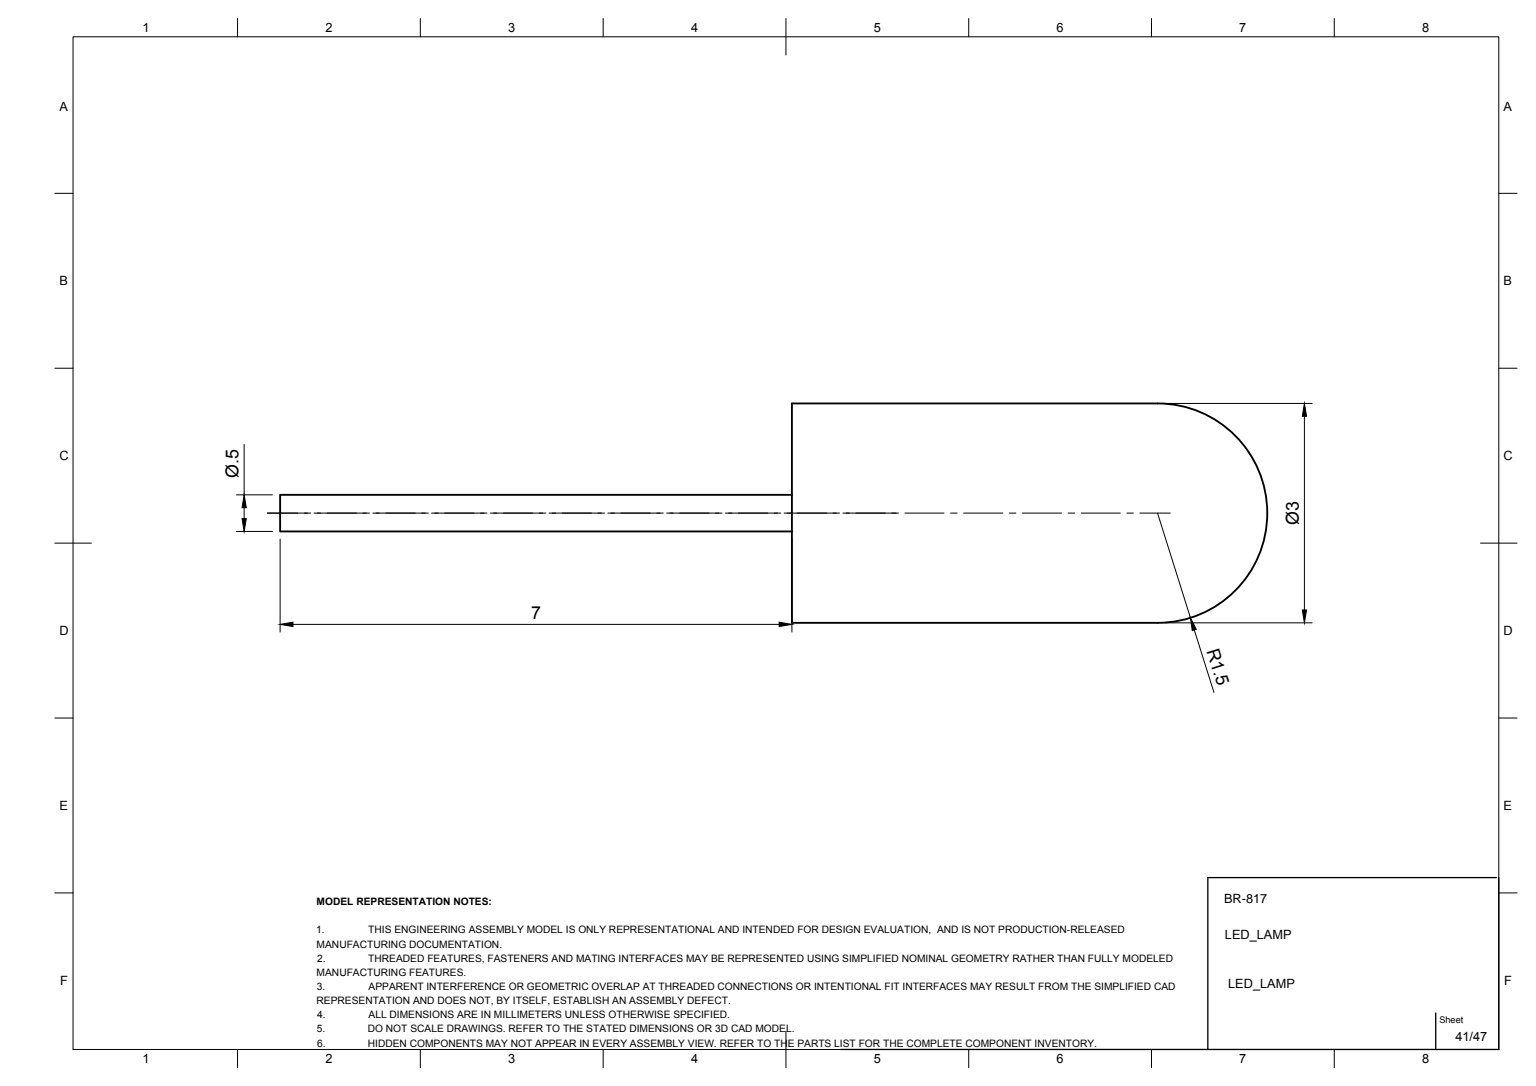
ISO-10303-21;
HEADER;
FILE_DESCRIPTION((''),'2;1');
FILE_NAME('LED_LAMP.step','2026-10-01T22:07:29-07:00',(''),(''),'','','');
FILE_SCHEMA (('AUTOMOTIVE_DESIGN { 1 0 10303 214 3 1 1 }'));
ENDSEC;
DATA;
#10=MECHANICAL_DESIGN_GEOMETRIC_PRESENTATION_REPRESENTATION('',(#572,#573,#574),#15484);
#291=SPHERICAL_SURFACE('',#9810,0.15) ;
#292=SPHERICAL_SURFACE('',#9813,0.15) ;
#501=SHAPE_REPRESENTATION_RELATIONSHIP('SRR','None',#15652,#536) ;
#536=ADVANCED_BREP_SHAPE_REPRESENTATION('',(#613,#614,#615),#15476) ;
#572=STYLED_ITEM('',(#15841),#613) ;
#573=STYLED_ITEM('',(#15842),#614) ;
#574=STYLED_ITEM('',(#15842),#615) ;
#613=MANIFOLD_SOLID_BREP('LED_BODY',#8283) ;
#614=MANIFOLD_SOLID_BREP('LED_LEADS',#8284) ;
#615=MANIFOLD_SOLID_BREP('LED_LEADS',#8285) ;
#795=CYLINDRICAL_SURFACE('',#9815,0.15) ;
#796=CYLINDRICAL_SURFACE('',#9818,0.025) ;
#797=CYLINDRICAL_SURFACE('',#9823,0.025) ;
#1329=CIRCLE('',#9811,0.15) ;
#1330=CIRCLE('',#9812,0.15) ;
#1331=CIRCLE('',#9814,0.15) ;
#1332=CIRCLE('',#9816,0.15) ;
#1333=CIRCLE('',#9819,0.025) ;
#1334=CIRCLE('',#9820,0.025) ;
#1335=CIRCLE('',#9824,0.025) ;
#1336=CIRCLE('',#9825,0.025) ;
#1812=FACE_OUTER_BOUND('',#2383,.T.) ;
#1813=FACE_OUTER_BOUND('',#2384,.T.) ;
#1814=FACE_OUTER_BOUND('',#2385,.T.) ;
#1815=FACE_OUTER_BOUND('',#2386,.T.) ;
#1816=FACE_OUTER_BOUND('',#2387,.T.) ;
#1817=FACE_OUTER_BOUND('',#2388,.T.) ;
#1818=FACE_OUTER_BOUND('',#2389,.T.) ;
#1819=FACE_OUTER_BOUND('',#2390,.T.) ;
#1820=FACE_OUTER_BOUND('',#2391,.T.) ;
#1821=FACE_OUTER_BOUND('',#2392,.T.) ;
#2383=EDGE_LOOP('',(#7377,#7378)) ;
#2384=EDGE_LOOP('',(#7379,#7380)) ;
#2385=EDGE_LOOP('',(#7381,#7382,#7383,#7384,#7385)) ;
#2386=EDGE_LOOP('',(#7386)) ;
#2387=EDGE_LOOP('',(#7387,#7388,#7389,#7390)) ;
#2388=EDGE_LOOP('',(#7391)) ;
#2389=EDGE_LOOP('',(#7392)) ;
#2390=EDGE_LOOP('',(#7393,#7394,#7395,#7396)) ;
#2391=EDGE_LOOP('',(#7397)) ;
#2392=EDGE_LOOP('',(#7398)) ;
#2870=LINE('',#15197,#3344) ;
#2871=LINE('',#15203,#3345) ;
#2872=LINE('',#15211,#3346) ;
#3344=VECTOR('',#12625,0.15) ;
#3345=VECTOR('',#12632,0.025) ;
#3346=VECTOR('',#12643,0.025) ;
#4088=VERTEX_POINT('',#15188) ;
#4089=VERTEX_POINT('',#15189) ;
#4090=VERTEX_POINT('',#15195) ;
#4091=VERTEX_POINT('',#15200) ;
#4092=VERTEX_POINT('',#15202) ;
#4093=VERTEX_POINT('',#15208) ;
#4094=VERTEX_POINT('',#15210) ;
#5193=EDGE_CURVE('',#4088,#4089,#1329,.T.) ;
#5194=EDGE_CURVE('',#4088,#4089,#1330,.T.) ;
#5195=EDGE_CURVE('',#4089,#4088,#1331,.T.) ;
#5196=EDGE_CURVE('',#4090,#4090,#1332,.T.) ;
#5197=EDGE_CURVE('',#4090,#4088,#2870,.T.) ;
#5198=EDGE_CURVE('',#4091,#4091,#1333,.T.) ;
#5199=EDGE_CURVE('',#4091,#4092,#2871,.T.) ;
#5200=EDGE_CURVE('',#4092,#4092,#1334,.T.) ;
#5201=EDGE_CURVE('',#4093,#4093,#1335,.T.) ;
#5202=EDGE_CURVE('',#4093,#4094,#2872,.T.) ;
#5203=EDGE_CURVE('',#4094,#4094,#1336,.T.) ;
#7377=ORIENTED_EDGE('',*,*,#5193,.F.) ;
#7378=ORIENTED_EDGE('',*,*,#5194,.T.) ;
#7379=ORIENTED_EDGE('',*,*,#5193,.T.) ;
#7380=ORIENTED_EDGE('',*,*,#5195,.T.) ;
#7381=ORIENTED_EDGE('',*,*,#5196,.F.) ;
#7382=ORIENTED_EDGE('',*,*,#5197,.T.) ;
#7383=ORIENTED_EDGE('',*,*,#5195,.F.) ;
#7384=ORIENTED_EDGE('',*,*,#5194,.F.) ;
#7385=ORIENTED_EDGE('',*,*,#5197,.F.) ;
#7386=ORIENTED_EDGE('',*,*,#5196,.T.) ;
#7387=ORIENTED_EDGE('',*,*,#5198,.F.) ;
#7388=ORIENTED_EDGE('',*,*,#5199,.T.) ;
#7389=ORIENTED_EDGE('',*,*,#5200,.F.) ;
#7390=ORIENTED_EDGE('',*,*,#5199,.F.) ;
#7391=ORIENTED_EDGE('',*,*,#5200,.T.) ;
#7392=ORIENTED_EDGE('',*,*,#5198,.T.) ;
#7393=ORIENTED_EDGE('',*,*,#5201,.F.) ;
#7394=ORIENTED_EDGE('',*,*,#5202,.T.) ;
#7395=ORIENTED_EDGE('',*,*,#5203,.F.) ;
#7396=ORIENTED_EDGE('',*,*,#5202,.F.) ;
#7397=ORIENTED_EDGE('',*,*,#5203,.T.) ;
#7398=ORIENTED_EDGE('',*,*,#5201,.T.) ;
#7716=PLANE('',#9817) ;
#7717=PLANE('',#9821) ;
#7718=PLANE('',#9822) ;
#7719=PLANE('',#9826) ;
#7720=PLANE('',#9827) ;
#8199=ADVANCED_FACE('',(#1812),#291,.T.) ;
#8200=ADVANCED_FACE('',(#1813),#292,.T.) ;
#8201=ADVANCED_FACE('',(#1814),#795,.T.) ;
#8202=ADVANCED_FACE('',(#1815),#7716,.T.) ;
#8203=ADVANCED_FACE('',(#1816),#796,.T.) ;
#8204=ADVANCED_FACE('',(#1817),#7717,.T.) ;
#8205=ADVANCED_FACE('',(#1818),#7718,.T.) ;
#8206=ADVANCED_FACE('',(#1819),#797,.T.) ;
#8207=ADVANCED_FACE('',(#1820),#7719,.T.) ;
#8208=ADVANCED_FACE('',(#1821),#7720,.T.) ;
#8283=CLOSED_SHELL('',(#8199,#8200,#8201,#8202)) ;
#8284=CLOSED_SHELL('',(#8203,#8204,#8205)) ;
#8285=CLOSED_SHELL('',(#8206,#8207,#8208)) ;
#9809=AXIS2_PLACEMENT_3D('',#15186,#12609,#12610) ;
#9810=AXIS2_PLACEMENT_3D('',#15187,#12611,#12612) ;
#9811=AXIS2_PLACEMENT_3D('',#15190,#12613,#12614) ;
#9812=AXIS2_PLACEMENT_3D('',#15191,#12615,#12616) ;
#9813=AXIS2_PLACEMENT_3D('',#15192,#12617,#12618) ;
#9814=AXIS2_PLACEMENT_3D('',#15193,#12619,#12620) ;
#9815=AXIS2_PLACEMENT_3D('',#15194,#12621,#12622) ;
#9816=AXIS2_PLACEMENT_3D('',#15196,#12623,#12624) ;
#9817=AXIS2_PLACEMENT_3D('',#15198,#12626,#12627) ;
#9818=AXIS2_PLACEMENT_3D('',#15199,#12628,#12629) ;
#9819=AXIS2_PLACEMENT_3D('',#15201,#12630,#12631) ;
#9820=AXIS2_PLACEMENT_3D('',#15204,#12633,#12634) ;
#9821=AXIS2_PLACEMENT_3D('',#15205,#12635,#12636) ;
#9822=AXIS2_PLACEMENT_3D('',#15206,#12637,#12638) ;
#9823=AXIS2_PLACEMENT_3D('',#15207,#12639,#12640) ;
#9824=AXIS2_PLACEMENT_3D('',#15209,#12641,#12642) ;
#9825=AXIS2_PLACEMENT_3D('',#15212,#12644,#12645) ;
#9826=AXIS2_PLACEMENT_3D('',#15213,#12646,#12647) ;
#9827=AXIS2_PLACEMENT_3D('',#15214,#12648,#12649) ;
#12609=DIRECTION('axis',(0.,0.,1.)) ;
#12610=DIRECTION('refdir',(1.,0.,0.)) ;
#12611=DIRECTION('center_axis',(0.,0.,1.)) ;
#12612=DIRECTION('ref_axis',(1.,0.,0.)) ;
#12613=DIRECTION('center_axis',(0.,-1.,0.)) ;
#12614=DIRECTION('ref_axis',(-1.,0.,0.)) ;
#12615=DIRECTION('center_axis',(-1.,0.,0.)) ;
#12616=DIRECTION('ref_axis',(0.,0.,-1.)) ;
#12617=DIRECTION('center_axis',(0.,0.,1.)) ;
#12618=DIRECTION('ref_axis',(1.,0.,0.)) ;
#12619=DIRECTION('center_axis',(-1.,0.,0.)) ;
#12620=DIRECTION('ref_axis',(0.,0.,-1.)) ;
#12621=DIRECTION('center_axis',(1.,0.,0.)) ;
#12622=DIRECTION('ref_axis',(0.,0.,-1.)) ;
#12623=DIRECTION('center_axis',(1.,0.,0.)) ;
#12624=DIRECTION('ref_axis',(0.,0.,-1.)) ;
#12625=DIRECTION('',(-1.,0.,0.)) ;
#12626=DIRECTION('center_axis',(1.,0.,0.)) ;
#12627=DIRECTION('ref_axis',(0.,0.,-1.)) ;
#12628=DIRECTION('center_axis',(1.,0.,0.)) ;
#12629=DIRECTION('ref_axis',(0.,0.,-1.)) ;
#12630=DIRECTION('center_axis',(1.,0.,0.)) ;
#12631=DIRECTION('ref_axis',(0.,0.,-1.)) ;
#12632=DIRECTION('',(-1.,0.,0.)) ;
#12633=DIRECTION('center_axis',(-1.,0.,0.)) ;
#12634=DIRECTION('ref_axis',(0.,0.,-1.)) ;
#12635=DIRECTION('center_axis',(-1.,0.,0.)) ;
#12636=DIRECTION('ref_axis',(0.,0.,1.)) ;
#12637=DIRECTION('center_axis',(1.,0.,0.)) ;
#12638=DIRECTION('ref_axis',(0.,0.,-1.)) ;
#12639=DIRECTION('center_axis',(1.,0.,0.)) ;
#12640=DIRECTION('ref_axis',(0.,0.,-1.)) ;
#12641=DIRECTION('center_axis',(1.,0.,0.)) ;
#12642=DIRECTION('ref_axis',(0.,0.,-1.)) ;
#12643=DIRECTION('',(-1.,0.,0.)) ;
#12644=DIRECTION('center_axis',(-1.,0.,0.)) ;
#12645=DIRECTION('ref_axis',(0.,0.,-1.)) ;
#12646=DIRECTION('center_axis',(-1.,0.,0.)) ;
#12647=DIRECTION('ref_axis',(0.,0.,1.)) ;
#12648=DIRECTION('center_axis',(1.,0.,0.)) ;
#12649=DIRECTION('ref_axis',(0.,0.,-1.)) ;
#15186=CARTESIAN_POINT('',(0.,0.,0.)) ;
#15187=CARTESIAN_POINT('Origin',(-3.4,-0.6,0.7)) ;
#15188=CARTESIAN_POINT('',(-3.4,-0.6,0.85)) ;
#15189=CARTESIAN_POINT('',(-3.4,-0.6,0.55)) ;
#15190=CARTESIAN_POINT('Origin',(-3.4,-0.6,0.7)) ;
#15191=CARTESIAN_POINT('Origin',(-3.4,-0.6,0.7)) ;
#15192=CARTESIAN_POINT('Origin',(-3.4,-0.6,0.7)) ;
#15193=CARTESIAN_POINT('Origin',(-3.4,-0.6,0.7)) ;
#15194=CARTESIAN_POINT('Origin',(-3.15,-0.6,0.7)) ;
#15195=CARTESIAN_POINT('',(-2.9,-0.6,0.85)) ;
#15196=CARTESIAN_POINT('Origin',(-2.9,-0.6,0.7)) ;
#15197=CARTESIAN_POINT('',(-3.15,-0.6,0.85)) ;
#15198=CARTESIAN_POINT('Origin',(-2.9,-0.6,0.7)) ;
#15199=CARTESIAN_POINT('Origin',(-2.55,-0.55,0.7)) ;
#15200=CARTESIAN_POINT('',(-2.2,-0.55,0.725)) ;
#15201=CARTESIAN_POINT('Origin',(-2.2,-0.55,0.7)) ;
#15202=CARTESIAN_POINT('',(-2.9,-0.55,0.725)) ;
#15203=CARTESIAN_POINT('',(-2.55,-0.55,0.725)) ;
#15204=CARTESIAN_POINT('Origin',(-2.9,-0.55,0.7)) ;
#15205=CARTESIAN_POINT('Origin',(-2.9,-0.55,0.7)) ;
#15206=CARTESIAN_POINT('Origin',(-2.2,-0.55,0.7)) ;
#15207=CARTESIAN_POINT('Origin',(-2.55,-0.65,0.7)) ;
#15208=CARTESIAN_POINT('',(-2.2,-0.65,0.725)) ;
#15209=CARTESIAN_POINT('Origin',(-2.2,-0.65,0.7)) ;
#15210=CARTESIAN_POINT('',(-2.9,-0.65,0.725)) ;
#15211=CARTESIAN_POINT('',(-2.55,-0.65,0.725)) ;
#15212=CARTESIAN_POINT('Origin',(-2.9,-0.65,0.7)) ;
#15213=CARTESIAN_POINT('Origin',(-2.9,-0.65,0.7)) ;
#15214=CARTESIAN_POINT('Origin',(-2.2,-0.65,0.7)) ;
#15433=UNCERTAINTY_MEASURE_WITH_UNIT(LENGTH_MEASURE(0.001),#15485,
'DISTANCE_ACCURACY_VALUE',
'Maximum model space distance between geometric entities at asserted c
onnectivities') ;
#15441=UNCERTAINTY_MEASURE_WITH_UNIT(LENGTH_MEASURE(0.001),#15485,
'DISTANCE_ACCURACY_VALUE',
'Maximum model space distance between geometric entities at asserted c
onnectivities') ;
#15476=(
GEOMETRIC_REPRESENTATION_CONTEXT(3)
GLOBAL_UNCERTAINTY_ASSIGNED_CONTEXT((#15433))
GLOBAL_UNIT_ASSIGNED_CONTEXT((#15485,#15487,#15488))
REPRESENTATION_CONTEXT('','3D')
) ;
#15484=(
GEOMETRIC_REPRESENTATION_CONTEXT(3)
GLOBAL_UNCERTAINTY_ASSIGNED_CONTEXT((#15441))
GLOBAL_UNIT_ASSIGNED_CONTEXT((#15485,#15487,#15488))
REPRESENTATION_CONTEXT('','3D')
) ;
#15485=(
LENGTH_UNIT()
NAMED_UNIT(*)
SI_UNIT(.CENTI.,.METRE.)
) ;
#15487=(
NAMED_UNIT(*)
PLANE_ANGLE_UNIT()
SI_UNIT($,.RADIAN.)
) ;
#15488=(
NAMED_UNIT(*)
SI_UNIT($,.STERADIAN.)
SOLID_ANGLE_UNIT()
) ;
#15523=SHAPE_DEFINITION_REPRESENTATION(#15591,#15652) ;
#15591=PRODUCT_DEFINITION_SHAPE('',$,#15695) ;
#15652=SHAPE_REPRESENTATION('',(#9809),#15476) ;
#15660=PRODUCT_DEFINITION_CONTEXT('part definition',#15788,'design') ;
#15695=PRODUCT_DEFINITION('LED_LAMP','LED_LAMP',#15737,#15660) ;
#15737=PRODUCT_DEFINITION_FORMATION('',$,#15824) ;
#15788=APPLICATION_CONTEXT(
'Core Data for Automotive Mechanical Design Process') ;
#15789=PRODUCT_CONTEXT('part definition',#15788,'mechanical') ;
#15824=PRODUCT('LED_LAMP','LED_LAMP',$,(#15789)) ;
#15841=PRESENTATION_STYLE_ASSIGNMENT((#15853)) ;
#15842=PRESENTATION_STYLE_ASSIGNMENT((#15854)) ;
#15853=SURFACE_STYLE_USAGE(.BOTH.,#15865) ;
#15854=SURFACE_STYLE_USAGE(.BOTH.,#15866) ;
#15865=SURFACE_SIDE_STYLE('',(#15877)) ;
#15866=SURFACE_SIDE_STYLE('',(#15878)) ;
#15877=SURFACE_STYLE_FILL_AREA(#15889) ;
#15878=SURFACE_STYLE_FILL_AREA(#15890) ;
#15889=FILL_AREA_STYLE('Plastic - Glossy (Grey)',(#15901)) ;
#15890=FILL_AREA_STYLE('Copper - Polished',(#15902)) ;
#15901=FILL_AREA_STYLE_COLOUR('Plastic - Glossy (Grey)',#15913) ;
#15902=FILL_AREA_STYLE_COLOUR('Copper - Polished',#15914) ;
#15913=COLOUR_RGB('Plastic - Glossy (Grey)', 0.09019608, 0.27058824, 0.51372549) ;
#15914=COLOUR_RGB('Copper - Polished', 0.66274510, 0.83137255, 0.94901961) ;
ENDSEC;
END-ISO-10303-21;
